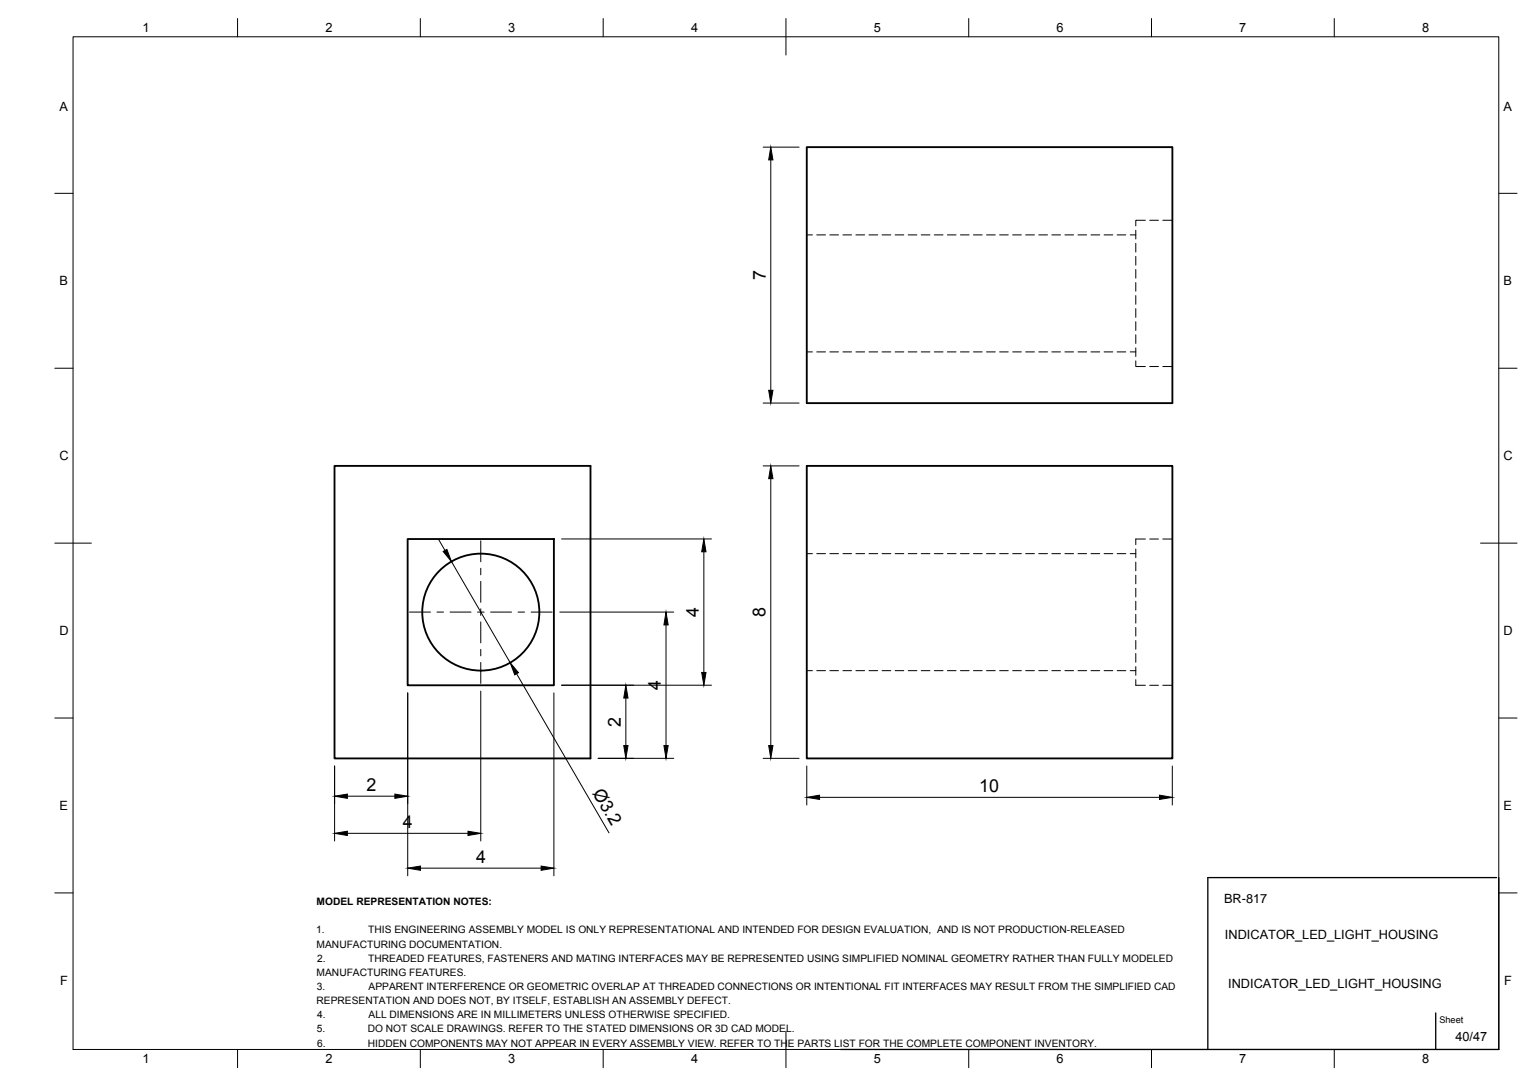
ISO-10303-21;
HEADER;
FILE_DESCRIPTION((''),'2;1');
FILE_NAME('INDICATOR_LED_LIGHT_HOUSING.step','2026-10-01T22:07:29-07:00',(''),(''),'','','');
FILE_SCHEMA (('AUTOMOTIVE_DESIGN { 1 0 10303 214 3 1 1 }'));
ENDSEC;
DATA;
#10=MECHANICAL_DESIGN_GEOMETRIC_PRESENTATION_REPRESENTATION('',(#571),#15484);
#500=SHAPE_REPRESENTATION_RELATIONSHIP('SRR','None',#15651,#535) ;
#535=ADVANCED_BREP_SHAPE_REPRESENTATION('',(#612),#15475) ;
#571=STYLED_ITEM('',(#15840),#612) ;
#612=MANIFOLD_SOLID_BREP('INDICATOR_LED_LIGHT_HOUSING',#8282) ;
#794=CYLINDRICAL_SURFACE('',#9801,0.16) ;
#878=FACE_BOUND('',#2373,.T.) ;
#879=FACE_BOUND('',#2379,.T.) ;
#880=FACE_BOUND('',#2382,.T.) ;
#1327=CIRCLE('',#9800,0.16) ;
#1328=CIRCLE('',#9802,0.16) ;
#1800=FACE_OUTER_BOUND('',#2368,.T.) ;
#1801=FACE_OUTER_BOUND('',#2369,.T.) ;
#1802=FACE_OUTER_BOUND('',#2370,.T.) ;
#1803=FACE_OUTER_BOUND('',#2371,.T.) ;
#1804=FACE_OUTER_BOUND('',#2372,.T.) ;
#1805=FACE_OUTER_BOUND('',#2374,.T.) ;
#1806=FACE_OUTER_BOUND('',#2375,.T.) ;
#1807=FACE_OUTER_BOUND('',#2376,.T.) ;
#1808=FACE_OUTER_BOUND('',#2377,.T.) ;
#1809=FACE_OUTER_BOUND('',#2378,.T.) ;
#1810=FACE_OUTER_BOUND('',#2380,.T.) ;
#1811=FACE_OUTER_BOUND('',#2381,.T.) ;
#2368=EDGE_LOOP('',(#7323,#7324,#7325,#7326)) ;
#2369=EDGE_LOOP('',(#7327,#7328,#7329,#7330)) ;
#2370=EDGE_LOOP('',(#7331,#7332,#7333,#7334)) ;
#2371=EDGE_LOOP('',(#7335,#7336,#7337,#7338)) ;
#2372=EDGE_LOOP('',(#7339,#7340,#7341,#7342)) ;
#2373=EDGE_LOOP('',(#7343)) ;
#2374=EDGE_LOOP('',(#7344,#7345,#7346,#7347)) ;
#2375=EDGE_LOOP('',(#7348,#7349,#7350,#7351)) ;
#2376=EDGE_LOOP('',(#7352,#7353,#7354,#7355)) ;
#2377=EDGE_LOOP('',(#7356,#7357,#7358,#7359)) ;
#2378=EDGE_LOOP('',(#7360,#7361,#7362,#7363)) ;
#2379=EDGE_LOOP('',(#7364,#7365,#7366,#7367)) ;
#2380=EDGE_LOOP('',(#7368,#7369,#7370,#7371)) ;
#2381=EDGE_LOOP('',(#7372,#7373,#7374,#7375)) ;
#2382=EDGE_LOOP('',(#7376)) ;
#2845=LINE('',#15132,#3319) ;
#2846=LINE('',#15134,#3320) ;
#2847=LINE('',#15136,#3321) ;
#2848=LINE('',#15137,#3322) ;
#2849=LINE('',#15140,#3323) ;
#2850=LINE('',#15142,#3324) ;
#2851=LINE('',#15143,#3325) ;
#2852=LINE('',#15146,#3326) ;
#2853=LINE('',#15148,#3327) ;
#2854=LINE('',#15149,#3328) ;
#2855=LINE('',#15151,#3329) ;
#2856=LINE('',#15152,#3330) ;
#2857=LINE('',#15158,#3331) ;
#2858=LINE('',#15163,#3332) ;
#2859=LINE('',#15165,#3333) ;
#2860=LINE('',#15167,#3334) ;
#2861=LINE('',#15168,#3335) ;
#2862=LINE('',#15172,#3336) ;
#2863=LINE('',#15174,#3337) ;
#2864=LINE('',#15176,#3338) ;
#2865=LINE('',#15177,#3339) ;
#2866=LINE('',#15179,#3340) ;
#2867=LINE('',#15180,#3341) ;
#2868=LINE('',#15182,#3342) ;
#2869=LINE('',#15184,#3343) ;
#3319=VECTOR('',#12558,1.) ;
#3320=VECTOR('',#12559,1.) ;
#3321=VECTOR('',#12560,1.) ;
#3322=VECTOR('',#12561,1.) ;
#3323=VECTOR('',#12564,1.) ;
#3324=VECTOR('',#12565,1.) ;
#3325=VECTOR('',#12566,1.) ;
#3326=VECTOR('',#12569,1.) ;
#3327=VECTOR('',#12570,1.) ;
#3328=VECTOR('',#12571,1.) ;
#3329=VECTOR('',#12574,1.) ;
#3330=VECTOR('',#12575,1.) ;
#3331=VECTOR('',#12582,0.16) ;
#3332=VECTOR('',#12587,1.) ;
#3333=VECTOR('',#12588,1.) ;
#3334=VECTOR('',#12589,1.) ;
#3335=VECTOR('',#12590,1.) ;
#3336=VECTOR('',#12593,1.) ;
#3337=VECTOR('',#12594,1.) ;
#3338=VECTOR('',#12595,1.) ;
#3339=VECTOR('',#12596,1.) ;
#3340=VECTOR('',#12599,1.) ;
#3341=VECTOR('',#12600,1.) ;
#3342=VECTOR('',#12603,1.) ;
#3343=VECTOR('',#12606,1.) ;
#4070=VERTEX_POINT('',#15130) ;
#4071=VERTEX_POINT('',#15131) ;
#4072=VERTEX_POINT('',#15133) ;
#4073=VERTEX_POINT('',#15135) ;
#4074=VERTEX_POINT('',#15139) ;
#4075=VERTEX_POINT('',#15141) ;
#4076=VERTEX_POINT('',#15145) ;
#4077=VERTEX_POINT('',#15147) ;
#4078=VERTEX_POINT('',#15154) ;
#4079=VERTEX_POINT('',#15157) ;
#4080=VERTEX_POINT('',#15161) ;
#4081=VERTEX_POINT('',#15162) ;
#4082=VERTEX_POINT('',#15164) ;
#4083=VERTEX_POINT('',#15166) ;
#4084=VERTEX_POINT('',#15170) ;
#4085=VERTEX_POINT('',#15171) ;
#4086=VERTEX_POINT('',#15173) ;
#4087=VERTEX_POINT('',#15175) ;
#5166=EDGE_CURVE('',#4070,#4071,#2845,.T.) ;
#5167=EDGE_CURVE('',#4072,#4070,#2846,.T.) ;
#5168=EDGE_CURVE('',#4073,#4072,#2847,.T.) ;
#5169=EDGE_CURVE('',#4071,#4073,#2848,.T.) ;
#5170=EDGE_CURVE('',#4071,#4074,#2849,.T.) ;
#5171=EDGE_CURVE('',#4073,#4075,#2850,.T.) ;
#5172=EDGE_CURVE('',#4075,#4074,#2851,.T.) ;
#5173=EDGE_CURVE('',#4074,#4076,#2852,.T.) ;
#5174=EDGE_CURVE('',#4077,#4075,#2853,.T.) ;
#5175=EDGE_CURVE('',#4076,#4077,#2854,.T.) ;
#5176=EDGE_CURVE('',#4076,#4070,#2855,.T.) ;
#5177=EDGE_CURVE('',#4072,#4077,#2856,.T.) ;
#5178=EDGE_CURVE('',#4078,#4078,#1327,.T.) ;
#5179=EDGE_CURVE('',#4078,#4079,#2857,.T.) ;
#5180=EDGE_CURVE('',#4079,#4079,#1328,.T.) ;
#5181=EDGE_CURVE('',#4080,#4081,#2858,.T.) ;
#5182=EDGE_CURVE('',#4081,#4082,#2859,.T.) ;
#5183=EDGE_CURVE('',#4082,#4083,#2860,.T.) ;
#5184=EDGE_CURVE('',#4083,#4080,#2861,.T.) ;
#5185=EDGE_CURVE('',#4084,#4085,#2862,.T.) ;
#5186=EDGE_CURVE('',#4085,#4086,#2863,.T.) ;
#5187=EDGE_CURVE('',#4086,#4087,#2864,.T.) ;
#5188=EDGE_CURVE('',#4087,#4084,#2865,.T.) ;
#5189=EDGE_CURVE('',#4083,#4086,#2866,.T.) ;
#5190=EDGE_CURVE('',#4080,#4085,#2867,.T.) ;
#5191=EDGE_CURVE('',#4082,#4087,#2868,.T.) ;
#5192=EDGE_CURVE('',#4081,#4084,#2869,.T.) ;
#7323=ORIENTED_EDGE('',*,*,#5166,.F.) ;
#7324=ORIENTED_EDGE('',*,*,#5167,.F.) ;
#7325=ORIENTED_EDGE('',*,*,#5168,.F.) ;
#7326=ORIENTED_EDGE('',*,*,#5169,.F.) ;
#7327=ORIENTED_EDGE('',*,*,#5170,.F.) ;
#7328=ORIENTED_EDGE('',*,*,#5169,.T.) ;
#7329=ORIENTED_EDGE('',*,*,#5171,.T.) ;
#7330=ORIENTED_EDGE('',*,*,#5172,.T.) ;
#7331=ORIENTED_EDGE('',*,*,#5173,.F.) ;
#7332=ORIENTED_EDGE('',*,*,#5172,.F.) ;
#7333=ORIENTED_EDGE('',*,*,#5174,.F.) ;
#7334=ORIENTED_EDGE('',*,*,#5175,.F.) ;
#7335=ORIENTED_EDGE('',*,*,#5176,.F.) ;
#7336=ORIENTED_EDGE('',*,*,#5175,.T.) ;
#7337=ORIENTED_EDGE('',*,*,#5177,.F.) ;
#7338=ORIENTED_EDGE('',*,*,#5167,.T.) ;
#7339=ORIENTED_EDGE('',*,*,#5171,.F.) ;
#7340=ORIENTED_EDGE('',*,*,#5168,.T.) ;
#7341=ORIENTED_EDGE('',*,*,#5177,.T.) ;
#7342=ORIENTED_EDGE('',*,*,#5174,.T.) ;
#7343=ORIENTED_EDGE('',*,*,#5178,.F.) ;
#7344=ORIENTED_EDGE('',*,*,#5178,.T.) ;
#7345=ORIENTED_EDGE('',*,*,#5179,.T.) ;
#7346=ORIENTED_EDGE('',*,*,#5180,.F.) ;
#7347=ORIENTED_EDGE('',*,*,#5179,.F.) ;
#7348=ORIENTED_EDGE('',*,*,#5181,.T.) ;
#7349=ORIENTED_EDGE('',*,*,#5182,.T.) ;
#7350=ORIENTED_EDGE('',*,*,#5183,.T.) ;
#7351=ORIENTED_EDGE('',*,*,#5184,.T.) ;
#7352=ORIENTED_EDGE('',*,*,#5185,.T.) ;
#7353=ORIENTED_EDGE('',*,*,#5186,.T.) ;
#7354=ORIENTED_EDGE('',*,*,#5187,.T.) ;
#7355=ORIENTED_EDGE('',*,*,#5188,.T.) ;
#7356=ORIENTED_EDGE('',*,*,#5189,.T.) ;
#7357=ORIENTED_EDGE('',*,*,#5186,.F.) ;
#7358=ORIENTED_EDGE('',*,*,#5190,.F.) ;
#7359=ORIENTED_EDGE('',*,*,#5184,.F.) ;
#7360=ORIENTED_EDGE('',*,*,#5191,.T.) ;
#7361=ORIENTED_EDGE('',*,*,#5187,.F.) ;
#7362=ORIENTED_EDGE('',*,*,#5189,.F.) ;
#7363=ORIENTED_EDGE('',*,*,#5183,.F.) ;
#7364=ORIENTED_EDGE('',*,*,#5173,.T.) ;
#7365=ORIENTED_EDGE('',*,*,#5176,.T.) ;
#7366=ORIENTED_EDGE('',*,*,#5166,.T.) ;
#7367=ORIENTED_EDGE('',*,*,#5170,.T.) ;
#7368=ORIENTED_EDGE('',*,*,#5192,.T.) ;
#7369=ORIENTED_EDGE('',*,*,#5188,.F.) ;
#7370=ORIENTED_EDGE('',*,*,#5191,.F.) ;
#7371=ORIENTED_EDGE('',*,*,#5182,.F.) ;
#7372=ORIENTED_EDGE('',*,*,#5190,.T.) ;
#7373=ORIENTED_EDGE('',*,*,#5185,.F.) ;
#7374=ORIENTED_EDGE('',*,*,#5192,.F.) ;
#7375=ORIENTED_EDGE('',*,*,#5181,.F.) ;
#7376=ORIENTED_EDGE('',*,*,#5180,.T.) ;
#7705=PLANE('',#9795) ;
#7706=PLANE('',#9796) ;
#7707=PLANE('',#9797) ;
#7708=PLANE('',#9798) ;
#7709=PLANE('',#9799) ;
#7710=PLANE('',#9803) ;
#7711=PLANE('',#9804) ;
#7712=PLANE('',#9805) ;
#7713=PLANE('',#9806) ;
#7714=PLANE('',#9807) ;
#7715=PLANE('',#9808) ;
#8187=ADVANCED_FACE('',(#1800),#7705,.F.) ;
#8188=ADVANCED_FACE('',(#1801),#7706,.T.) ;
#8189=ADVANCED_FACE('',(#1802),#7707,.T.) ;
#8190=ADVANCED_FACE('',(#1803),#7708,.T.) ;
#8191=ADVANCED_FACE('',(#1804,#878),#7709,.T.) ;
#8192=ADVANCED_FACE('',(#1805),#794,.F.) ;
#8193=ADVANCED_FACE('',(#1806),#7710,.T.) ;
#8194=ADVANCED_FACE('',(#1807),#7711,.F.) ;
#8195=ADVANCED_FACE('',(#1808),#7712,.F.) ;
#8196=ADVANCED_FACE('',(#1809,#879),#7713,.F.) ;
#8197=ADVANCED_FACE('',(#1810),#7714,.F.) ;
#8198=ADVANCED_FACE('',(#1811,#880),#7715,.F.) ;
#8282=CLOSED_SHELL('',(#8187,#8188,#8189,#8190,#8191,#8192,#8193,#8194,
#8195,#8196,#8197,#8198)) ;
#9794=AXIS2_PLACEMENT_3D('',#15128,#12554,#12555) ;
#9795=AXIS2_PLACEMENT_3D('',#15129,#12556,#12557) ;
#9796=AXIS2_PLACEMENT_3D('',#15138,#12562,#12563) ;
#9797=AXIS2_PLACEMENT_3D('',#15144,#12567,#12568) ;
#9798=AXIS2_PLACEMENT_3D('',#15150,#12572,#12573) ;
#9799=AXIS2_PLACEMENT_3D('',#15153,#12576,#12577) ;
#9800=AXIS2_PLACEMENT_3D('',#15155,#12578,#12579) ;
#9801=AXIS2_PLACEMENT_3D('',#15156,#12580,#12581) ;
#9802=AXIS2_PLACEMENT_3D('',#15159,#12583,#12584) ;
#9803=AXIS2_PLACEMENT_3D('',#15160,#12585,#12586) ;
#9804=AXIS2_PLACEMENT_3D('',#15169,#12591,#12592) ;
#9805=AXIS2_PLACEMENT_3D('',#15178,#12597,#12598) ;
#9806=AXIS2_PLACEMENT_3D('',#15181,#12601,#12602) ;
#9807=AXIS2_PLACEMENT_3D('',#15183,#12604,#12605) ;
#9808=AXIS2_PLACEMENT_3D('',#15185,#12607,#12608) ;
#12554=DIRECTION('axis',(0.,0.,1.)) ;
#12555=DIRECTION('refdir',(1.,0.,0.)) ;
#12556=DIRECTION('center_axis',(0.,0.,1.)) ;
#12557=DIRECTION('ref_axis',(1.,0.,0.)) ;
#12558=DIRECTION('',(0.,-1.,0.)) ;
#12559=DIRECTION('',(-1.,0.,0.)) ;
#12560=DIRECTION('',(0.,1.,0.)) ;
#12561=DIRECTION('',(1.,0.,0.)) ;
#12562=DIRECTION('center_axis',(0.,1.,0.)) ;
#12563=DIRECTION('ref_axis',(0.,0.,1.)) ;
#12564=DIRECTION('',(0.,0.,-1.)) ;
#12565=DIRECTION('',(0.,0.,-1.)) ;
#12566=DIRECTION('',(-1.,0.,0.)) ;
#12567=DIRECTION('center_axis',(0.,0.,1.)) ;
#12568=DIRECTION('ref_axis',(1.,0.,0.)) ;
#12569=DIRECTION('',(0.,1.,0.)) ;
#12570=DIRECTION('',(0.,-1.,0.)) ;
#12571=DIRECTION('',(1.,0.,0.)) ;
#12572=DIRECTION('center_axis',(0.,-1.,0.)) ;
#12573=DIRECTION('ref_axis',(0.,0.,-1.)) ;
#12574=DIRECTION('',(0.,0.,1.)) ;
#12575=DIRECTION('',(0.,0.,-1.)) ;
#12576=DIRECTION('center_axis',(-1.,0.,0.)) ;
#12577=DIRECTION('ref_axis',(0.,0.,1.)) ;
#12578=DIRECTION('center_axis',(-1.,0.,0.)) ;
#12579=DIRECTION('ref_axis',(0.,0.,-1.)) ;
#12580=DIRECTION('center_axis',(1.,0.,0.)) ;
#12581=DIRECTION('ref_axis',(0.,0.,-1.)) ;
#12582=DIRECTION('',(1.,0.,0.)) ;
#12583=DIRECTION('center_axis',(-1.,0.,0.)) ;
#12584=DIRECTION('ref_axis',(0.,0.,-1.)) ;
#12585=DIRECTION('center_axis',(0.,0.,1.)) ;
#12586=DIRECTION('ref_axis',(1.,0.,0.)) ;
#12587=DIRECTION('',(0.,1.,0.)) ;
#12588=DIRECTION('',(-1.,0.,0.)) ;
#12589=DIRECTION('',(0.,-1.,0.)) ;
#12590=DIRECTION('',(1.,0.,0.)) ;
#12591=DIRECTION('center_axis',(0.,0.,1.)) ;
#12592=DIRECTION('ref_axis',(1.,0.,0.)) ;
#12593=DIRECTION('',(0.,-1.,0.)) ;
#12594=DIRECTION('',(-1.,0.,0.)) ;
#12595=DIRECTION('',(0.,1.,0.)) ;
#12596=DIRECTION('',(1.,0.,0.)) ;
#12597=DIRECTION('center_axis',(0.,1.,0.)) ;
#12598=DIRECTION('ref_axis',(0.,0.,1.)) ;
#12599=DIRECTION('',(0.,0.,-1.)) ;
#12600=DIRECTION('',(0.,0.,-1.)) ;
#12601=DIRECTION('center_axis',(1.,0.,0.)) ;
#12602=DIRECTION('ref_axis',(0.,0.,-1.)) ;
#12603=DIRECTION('',(0.,0.,-1.)) ;
#12604=DIRECTION('center_axis',(0.,-1.,0.)) ;
#12605=DIRECTION('ref_axis',(0.,0.,-1.)) ;
#12606=DIRECTION('',(0.,0.,-1.)) ;
#12607=DIRECTION('center_axis',(-1.,0.,0.)) ;
#12608=DIRECTION('ref_axis',(0.,0.,1.)) ;
#15128=CARTESIAN_POINT('',(0.,0.,0.)) ;
#15129=CARTESIAN_POINT('Origin',(-3.6,-0.6,0.9)) ;
#15130=CARTESIAN_POINT('',(-3.6,-0.4,0.9)) ;
#15131=CARTESIAN_POINT('',(-3.6,-0.8,0.9)) ;
#15132=CARTESIAN_POINT('',(-3.6,-0.6,0.9)) ;
#15133=CARTESIAN_POINT('',(-3.5,-0.4,0.9)) ;
#15134=CARTESIAN_POINT('',(-3.6,-0.4,0.9)) ;
#15135=CARTESIAN_POINT('',(-3.5,-0.8,0.9)) ;
#15136=CARTESIAN_POINT('',(-3.5,-0.6,0.9)) ;
#15137=CARTESIAN_POINT('',(-3.6,-0.8,0.9)) ;
#15138=CARTESIAN_POINT('Origin',(-3.6,-0.8,0.7)) ;
#15139=CARTESIAN_POINT('',(-3.6,-0.8,0.5)) ;
#15140=CARTESIAN_POINT('',(-3.6,-0.8,0.675)) ;
#15141=CARTESIAN_POINT('',(-3.5,-0.8,0.5)) ;
#15142=CARTESIAN_POINT('',(-3.5,-0.8,0.7)) ;
#15143=CARTESIAN_POINT('',(-3.6,-0.8,0.5)) ;
#15144=CARTESIAN_POINT('Origin',(-3.6,-0.6,0.5)) ;
#15145=CARTESIAN_POINT('',(-3.6,-0.4,0.5)) ;
#15146=CARTESIAN_POINT('',(-3.6,-0.6,0.5)) ;
#15147=CARTESIAN_POINT('',(-3.5,-0.4,0.5)) ;
#15148=CARTESIAN_POINT('',(-3.5,-0.6,0.5)) ;
#15149=CARTESIAN_POINT('',(-3.6,-0.4,0.5)) ;
#15150=CARTESIAN_POINT('Origin',(-3.6,-0.4,0.7)) ;
#15151=CARTESIAN_POINT('',(-3.6,-0.4,0.675)) ;
#15152=CARTESIAN_POINT('',(-3.5,-0.4,0.7)) ;
#15153=CARTESIAN_POINT('Origin',(-3.5,-0.6,0.7)) ;
#15154=CARTESIAN_POINT('',(-3.5,-0.6,0.86)) ;
#15155=CARTESIAN_POINT('Origin',(-3.5,-0.6,0.7)) ;
#15156=CARTESIAN_POINT('Origin',(-3.1,-0.6,0.7)) ;
#15157=CARTESIAN_POINT('',(-2.6,-0.6,0.86)) ;
#15158=CARTESIAN_POINT('',(-3.1,-0.6,0.86)) ;
#15159=CARTESIAN_POINT('Origin',(-2.6,-0.6,0.7)) ;
#15160=CARTESIAN_POINT('Origin',(-3.1,-0.6,1.)) ;
#15161=CARTESIAN_POINT('',(-2.6,-1.,1.)) ;
#15162=CARTESIAN_POINT('',(-2.6,-0.2,1.)) ;
#15163=CARTESIAN_POINT('',(-2.6,-0.6,1.)) ;
#15164=CARTESIAN_POINT('',(-3.6,-0.2,1.)) ;
#15165=CARTESIAN_POINT('',(-3.1,-0.2,1.)) ;
#15166=CARTESIAN_POINT('',(-3.6,-1.,1.)) ;
#15167=CARTESIAN_POINT('',(-3.6,-0.6,1.)) ;
#15168=CARTESIAN_POINT('',(-3.1,-1.,1.)) ;
#15169=CARTESIAN_POINT('Origin',(-3.1,-0.6,0.3)) ;
#15170=CARTESIAN_POINT('',(-2.6,-0.2,0.3)) ;
#15171=CARTESIAN_POINT('',(-2.6,-1.,0.3)) ;
#15172=CARTESIAN_POINT('',(-2.6,-0.6,0.3)) ;
#15173=CARTESIAN_POINT('',(-3.6,-1.,0.3)) ;
#15174=CARTESIAN_POINT('',(-3.1,-1.,0.3)) ;
#15175=CARTESIAN_POINT('',(-3.6,-0.2,0.3)) ;
#15176=CARTESIAN_POINT('',(-3.6,-0.6,0.3)) ;
#15177=CARTESIAN_POINT('',(-3.1,-0.2,0.3)) ;
#15178=CARTESIAN_POINT('Origin',(-3.1,-1.,0.65)) ;
#15179=CARTESIAN_POINT('',(-3.6,-1.,0.65)) ;
#15180=CARTESIAN_POINT('',(-2.6,-1.,0.65)) ;
#15181=CARTESIAN_POINT('Origin',(-3.6,-0.6,0.65)) ;
#15182=CARTESIAN_POINT('',(-3.6,-0.2,0.65)) ;
#15183=CARTESIAN_POINT('Origin',(-3.1,-0.2,0.65)) ;
#15184=CARTESIAN_POINT('',(-2.6,-0.2,0.65)) ;
#15185=CARTESIAN_POINT('Origin',(-2.6,-0.6,0.65)) ;
#15432=UNCERTAINTY_MEASURE_WITH_UNIT(LENGTH_MEASURE(0.001),#15485,
'DISTANCE_ACCURACY_VALUE',
'Maximum model space distance between geometric entities at asserted c
onnectivities') ;
#15441=UNCERTAINTY_MEASURE_WITH_UNIT(LENGTH_MEASURE(0.001),#15485,
'DISTANCE_ACCURACY_VALUE',
'Maximum model space distance between geometric entities at asserted c
onnectivities') ;
#15475=(
GEOMETRIC_REPRESENTATION_CONTEXT(3)
GLOBAL_UNCERTAINTY_ASSIGNED_CONTEXT((#15432))
GLOBAL_UNIT_ASSIGNED_CONTEXT((#15485,#15487,#15488))
REPRESENTATION_CONTEXT('','3D')
) ;
#15484=(
GEOMETRIC_REPRESENTATION_CONTEXT(3)
GLOBAL_UNCERTAINTY_ASSIGNED_CONTEXT((#15441))
GLOBAL_UNIT_ASSIGNED_CONTEXT((#15485,#15487,#15488))
REPRESENTATION_CONTEXT('','3D')
) ;
#15485=(
LENGTH_UNIT()
NAMED_UNIT(*)
SI_UNIT(.CENTI.,.METRE.)
) ;
#15487=(
NAMED_UNIT(*)
PLANE_ANGLE_UNIT()
SI_UNIT($,.RADIAN.)
) ;
#15488=(
NAMED_UNIT(*)
SI_UNIT($,.STERADIAN.)
SOLID_ANGLE_UNIT()
) ;
#15522=SHAPE_DEFINITION_REPRESENTATION(#15590,#15651) ;
#15590=PRODUCT_DEFINITION_SHAPE('',$,#15694) ;
#15651=SHAPE_REPRESENTATION('',(#9794),#15475) ;
#15660=PRODUCT_DEFINITION_CONTEXT('part definition',#15788,'design') ;
#15694=PRODUCT_DEFINITION('INDICATOR_LED_LIGHT_HOUSING',
'INDICATOR_LED_LIGHT_HOUSING',#15736,#15660) ;
#15736=PRODUCT_DEFINITION_FORMATION('',$,#15823) ;
#15788=APPLICATION_CONTEXT(
'Core Data for Automotive Mechanical Design Process') ;
#15789=PRODUCT_CONTEXT('part definition',#15788,'mechanical') ;
#15823=PRODUCT('INDICATOR_LED_LIGHT_HOUSING','INDICATOR_LED_LIGHT_HOUSING',
$,(#15789)) ;
#15840=PRESENTATION_STYLE_ASSIGNMENT((#15852)) ;
#15852=SURFACE_STYLE_USAGE(.BOTH.,#15864) ;
#15864=SURFACE_SIDE_STYLE('',(#15876)) ;
#15876=SURFACE_STYLE_FILL_AREA(#15888) ;
#15888=FILL_AREA_STYLE('Polycarbonate (Clear)',(#15900)) ;
#15900=FILL_AREA_STYLE_COLOUR('Polycarbonate (Clear)',#15912) ;
#15912=COLOUR_RGB('Polycarbonate (Clear)', 0.08235294, 0.09019608, 0.10196078) ;
ENDSEC;
END-ISO-10303-21;
